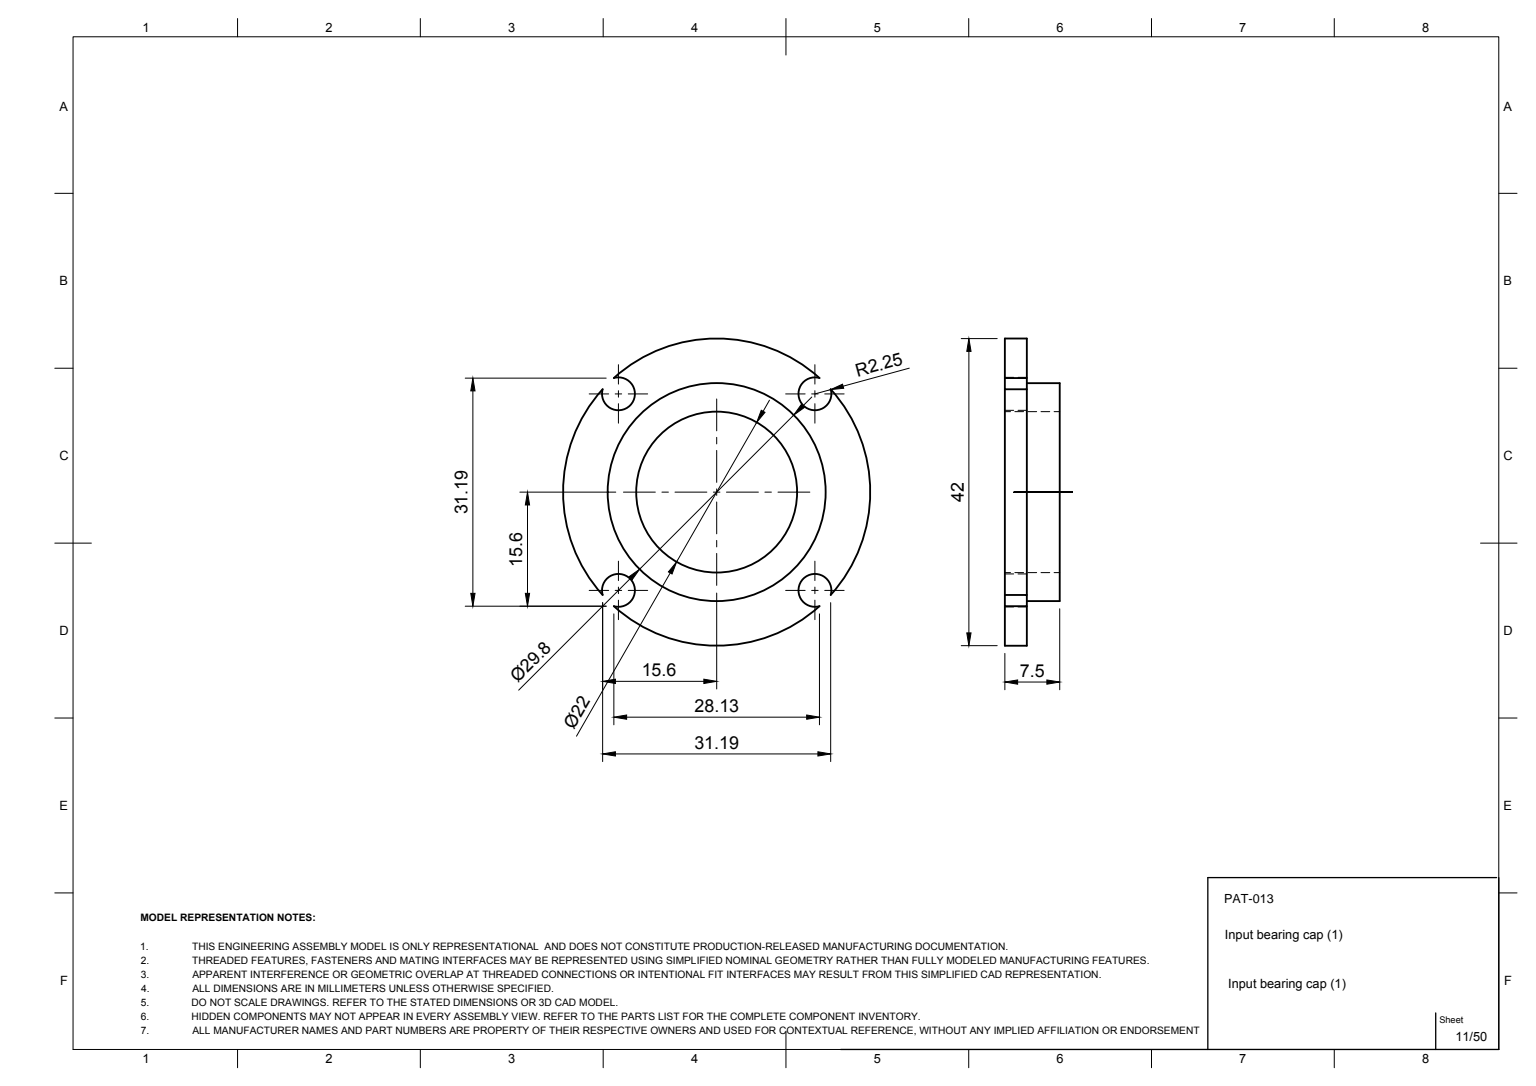
ISO-10303-21;
HEADER;
/* Generated by software containing ST-Developer
 * from STEP Tools, Inc. (www.steptools.com) 
 */

FILE_DESCRIPTION(
/* description */ ('Belt-driven linear axis on 2020 extrusion'),
/* implementation_level */ '2;1');

FILE_NAME(
/* name */ 'Input bearing cap (1).step',
/* time_stamp */ '2026-10-28T03:26:09-07:00',
/* author */ (''),
/* organization */ (''),
/* preprocessor_version */ 'ST-DEVELOPER v20.2',
/* originating_system */ 'Autodesk Translation Framework v15.17.0.0',
/* authorisation */ '');

FILE_SCHEMA (('AUTOMOTIVE_DESIGN { 1 0 10303 214 3 1 1 }'));
ENDSEC;

DATA;
#10=MECHANICAL_DESIGN_GEOMETRIC_PRESENTATION_REPRESENTATION('',(#618),#20096);
#524=SHAPE_REPRESENTATION_RELATIONSHIP('SRR','None',#20320,#570);
#570=ADVANCED_BREP_SHAPE_REPRESENTATION('',(#674),#20051);
#618=STYLED_ITEM('',(#20650),#674);
#674=MANIFOLD_SOLID_BREP('Body1',#10931);
#765=FACE_BOUND('',#2026,.T.);
#766=FACE_BOUND('',#2033,.T.);
#767=FACE_BOUND('',#2036,.T.);
#950=PLANE('',#11695);
#951=PLANE('',#11711);
#952=PLANE('',#11715);
#1352=FACE_OUTER_BOUND('',#2021,.T.);
#1353=FACE_OUTER_BOUND('',#2022,.T.);
#1354=FACE_OUTER_BOUND('',#2023,.T.);
#1355=FACE_OUTER_BOUND('',#2024,.T.);
#1356=FACE_OUTER_BOUND('',#2025,.T.);
#1357=FACE_OUTER_BOUND('',#2027,.T.);
#1358=FACE_OUTER_BOUND('',#2028,.T.);
#1359=FACE_OUTER_BOUND('',#2029,.T.);
#1360=FACE_OUTER_BOUND('',#2030,.T.);
#1361=FACE_OUTER_BOUND('',#2031,.T.);
#1362=FACE_OUTER_BOUND('',#2032,.T.);
#1363=FACE_OUTER_BOUND('',#2034,.T.);
#1364=FACE_OUTER_BOUND('',#2035,.T.);
#2021=EDGE_LOOP('',(#7667,#7668,#7669,#7670));
#2022=EDGE_LOOP('',(#7671,#7672,#7673,#7674));
#2023=EDGE_LOOP('',(#7675,#7676,#7677,#7678));
#2024=EDGE_LOOP('',(#7679,#7680,#7681,#7682));
#2025=EDGE_LOOP('',(#7683,#7684,#7685,#7686,#7687,#7688,#7689,#7690));
#2026=EDGE_LOOP('',(#7691));
#2027=EDGE_LOOP('',(#7692,#7693,#7694,#7695));
#2028=EDGE_LOOP('',(#7696,#7697,#7698,#7699));
#2029=EDGE_LOOP('',(#7700,#7701,#7702,#7703));
#2030=EDGE_LOOP('',(#7704,#7705,#7706,#7707));
#2031=EDGE_LOOP('',(#7708,#7709,#7710,#7711));
#2032=EDGE_LOOP('',(#7712));
#2033=EDGE_LOOP('',(#7713));
#2034=EDGE_LOOP('',(#7714,#7715,#7716,#7717));
#2035=EDGE_LOOP('',(#7718,#7719,#7720,#7721,#7722,#7723,#7724,#7725));
#2036=EDGE_LOOP('',(#7726));
#2790=LINE('',#16691,#3647);
#2791=LINE('',#16695,#3648);
#2792=LINE('',#16700,#3649);
#2793=LINE('',#16704,#3650);
#2794=LINE('',#16709,#3651);
#2795=LINE('',#16713,#3652);
#2796=LINE('',#16718,#3653);
#2797=LINE('',#16722,#3654);
#2798=LINE('',#16741,#3655);
#2799=LINE('',#16749,#3656);
#3647=VECTOR('',#13298,1.);
#3648=VECTOR('',#13301,1.);
#3649=VECTOR('',#13306,1.);
#3650=VECTOR('',#13309,1.);
#3651=VECTOR('',#13314,1.);
#3652=VECTOR('',#13317,1.);
#3653=VECTOR('',#13322,1.);
#3654=VECTOR('',#13325,1.);
#3655=VECTOR('',#13358,1.49);
#3656=VECTOR('',#13369,1.1);
#4461=CIRCLE('',#11684,0.225);
#4462=CIRCLE('',#11685,0.225);
#4463=CIRCLE('',#11687,0.225);
#4464=CIRCLE('',#11688,0.225);
#4465=CIRCLE('',#11690,0.225);
#4466=CIRCLE('',#11691,0.225);
#4467=CIRCLE('',#11693,0.225);
#4468=CIRCLE('',#11694,0.225);
#4469=CIRCLE('',#11696,2.1);
#4470=CIRCLE('',#11697,2.1);
#4471=CIRCLE('',#11698,2.1);
#4472=CIRCLE('',#11699,2.1);
#4473=CIRCLE('',#11700,1.49);
#4474=CIRCLE('',#11702,2.1);
#4475=CIRCLE('',#11704,2.1);
#4476=CIRCLE('',#11706,2.1);
#4477=CIRCLE('',#11708,2.1);
#4478=CIRCLE('',#11710,1.49);
#4479=CIRCLE('',#11712,1.1);
#4480=CIRCLE('',#11714,1.1);
#5030=VERTEX_POINT('',#16689);
#5031=VERTEX_POINT('',#16690);
#5032=VERTEX_POINT('',#16692);
#5033=VERTEX_POINT('',#16694);
#5034=VERTEX_POINT('',#16698);
#5035=VERTEX_POINT('',#16699);
#5036=VERTEX_POINT('',#16701);
#5037=VERTEX_POINT('',#16703);
#5038=VERTEX_POINT('',#16707);
#5039=VERTEX_POINT('',#16708);
#5040=VERTEX_POINT('',#16710);
#5041=VERTEX_POINT('',#16712);
#5042=VERTEX_POINT('',#16716);
#5043=VERTEX_POINT('',#16717);
#5044=VERTEX_POINT('',#16719);
#5045=VERTEX_POINT('',#16721);
#5046=VERTEX_POINT('',#16729);
#5047=VERTEX_POINT('',#16740);
#5048=VERTEX_POINT('',#16744);
#5049=VERTEX_POINT('',#16747);
#6048=EDGE_CURVE('',#5030,#5031,#2790,.T.);
#6049=EDGE_CURVE('',#5032,#5030,#4461,.T.);
#6050=EDGE_CURVE('',#5033,#5032,#2791,.T.);
#6051=EDGE_CURVE('',#5031,#5033,#4462,.T.);
#6052=EDGE_CURVE('',#5034,#5035,#2792,.T.);
#6053=EDGE_CURVE('',#5036,#5034,#4463,.T.);
#6054=EDGE_CURVE('',#5037,#5036,#2793,.T.);
#6055=EDGE_CURVE('',#5035,#5037,#4464,.T.);
#6056=EDGE_CURVE('',#5038,#5039,#2794,.T.);
#6057=EDGE_CURVE('',#5040,#5038,#4465,.T.);
#6058=EDGE_CURVE('',#5041,#5040,#2795,.T.);
#6059=EDGE_CURVE('',#5039,#5041,#4466,.T.);
#6060=EDGE_CURVE('',#5042,#5043,#2796,.T.);
#6061=EDGE_CURVE('',#5044,#5042,#4467,.T.);
#6062=EDGE_CURVE('',#5045,#5044,#2797,.T.);
#6063=EDGE_CURVE('',#5043,#5045,#4468,.T.);
#6064=EDGE_CURVE('',#5044,#5030,#4469,.T.);
#6065=EDGE_CURVE('',#5040,#5042,#4470,.T.);
#6066=EDGE_CURVE('',#5036,#5038,#4471,.T.);
#6067=EDGE_CURVE('',#5032,#5034,#4472,.T.);
#6068=EDGE_CURVE('',#5046,#5046,#4473,.T.);
#6069=EDGE_CURVE('',#5041,#5043,#4474,.T.);
#6070=EDGE_CURVE('',#5037,#5039,#4475,.T.);
#6071=EDGE_CURVE('',#5045,#5031,#4476,.T.);
#6072=EDGE_CURVE('',#5033,#5035,#4477,.T.);
#6073=EDGE_CURVE('',#5046,#5047,#2798,.T.);
#6074=EDGE_CURVE('',#5047,#5047,#4478,.T.);
#6075=EDGE_CURVE('',#5048,#5048,#4479,.T.);
#6076=EDGE_CURVE('',#5049,#5049,#4480,.T.);
#6077=EDGE_CURVE('',#5049,#5048,#2799,.T.);
#7667=ORIENTED_EDGE('',*,*,#6048,.F.);
#7668=ORIENTED_EDGE('',*,*,#6049,.F.);
#7669=ORIENTED_EDGE('',*,*,#6050,.F.);
#7670=ORIENTED_EDGE('',*,*,#6051,.F.);
#7671=ORIENTED_EDGE('',*,*,#6052,.F.);
#7672=ORIENTED_EDGE('',*,*,#6053,.F.);
#7673=ORIENTED_EDGE('',*,*,#6054,.F.);
#7674=ORIENTED_EDGE('',*,*,#6055,.F.);
#7675=ORIENTED_EDGE('',*,*,#6056,.F.);
#7676=ORIENTED_EDGE('',*,*,#6057,.F.);
#7677=ORIENTED_EDGE('',*,*,#6058,.F.);
#7678=ORIENTED_EDGE('',*,*,#6059,.F.);
#7679=ORIENTED_EDGE('',*,*,#6060,.F.);
#7680=ORIENTED_EDGE('',*,*,#6061,.F.);
#7681=ORIENTED_EDGE('',*,*,#6062,.F.);
#7682=ORIENTED_EDGE('',*,*,#6063,.F.);
#7683=ORIENTED_EDGE('',*,*,#6049,.T.);
#7684=ORIENTED_EDGE('',*,*,#6064,.F.);
#7685=ORIENTED_EDGE('',*,*,#6061,.T.);
#7686=ORIENTED_EDGE('',*,*,#6065,.F.);
#7687=ORIENTED_EDGE('',*,*,#6057,.T.);
#7688=ORIENTED_EDGE('',*,*,#6066,.F.);
#7689=ORIENTED_EDGE('',*,*,#6053,.T.);
#7690=ORIENTED_EDGE('',*,*,#6067,.F.);
#7691=ORIENTED_EDGE('',*,*,#6068,.T.);
#7692=ORIENTED_EDGE('',*,*,#6058,.T.);
#7693=ORIENTED_EDGE('',*,*,#6065,.T.);
#7694=ORIENTED_EDGE('',*,*,#6060,.T.);
#7695=ORIENTED_EDGE('',*,*,#6069,.F.);
#7696=ORIENTED_EDGE('',*,*,#6054,.T.);
#7697=ORIENTED_EDGE('',*,*,#6066,.T.);
#7698=ORIENTED_EDGE('',*,*,#6056,.T.);
#7699=ORIENTED_EDGE('',*,*,#6070,.F.);
#7700=ORIENTED_EDGE('',*,*,#6048,.T.);
#7701=ORIENTED_EDGE('',*,*,#6071,.F.);
#7702=ORIENTED_EDGE('',*,*,#6062,.T.);
#7703=ORIENTED_EDGE('',*,*,#6064,.T.);
#7704=ORIENTED_EDGE('',*,*,#6050,.T.);
#7705=ORIENTED_EDGE('',*,*,#6067,.T.);
#7706=ORIENTED_EDGE('',*,*,#6052,.T.);
#7707=ORIENTED_EDGE('',*,*,#6072,.F.);
#7708=ORIENTED_EDGE('',*,*,#6068,.F.);
#7709=ORIENTED_EDGE('',*,*,#6073,.T.);
#7710=ORIENTED_EDGE('',*,*,#6074,.T.);
#7711=ORIENTED_EDGE('',*,*,#6073,.F.);
#7712=ORIENTED_EDGE('',*,*,#6074,.F.);
#7713=ORIENTED_EDGE('',*,*,#6075,.F.);
#7714=ORIENTED_EDGE('',*,*,#6076,.F.);
#7715=ORIENTED_EDGE('',*,*,#6077,.T.);
#7716=ORIENTED_EDGE('',*,*,#6075,.T.);
#7717=ORIENTED_EDGE('',*,*,#6077,.F.);
#7718=ORIENTED_EDGE('',*,*,#6051,.T.);
#7719=ORIENTED_EDGE('',*,*,#6072,.T.);
#7720=ORIENTED_EDGE('',*,*,#6055,.T.);
#7721=ORIENTED_EDGE('',*,*,#6070,.T.);
#7722=ORIENTED_EDGE('',*,*,#6059,.T.);
#7723=ORIENTED_EDGE('',*,*,#6069,.T.);
#7724=ORIENTED_EDGE('',*,*,#6063,.T.);
#7725=ORIENTED_EDGE('',*,*,#6071,.T.);
#7726=ORIENTED_EDGE('',*,*,#6076,.T.);
#10118=CYLINDRICAL_SURFACE('',#11683,0.225);
#10119=CYLINDRICAL_SURFACE('',#11686,0.225);
#10120=CYLINDRICAL_SURFACE('',#11689,0.225);
#10121=CYLINDRICAL_SURFACE('',#11692,0.225);
#10122=CYLINDRICAL_SURFACE('',#11701,2.1);
#10123=CYLINDRICAL_SURFACE('',#11703,2.1);
#10124=CYLINDRICAL_SURFACE('',#11705,2.1);
#10125=CYLINDRICAL_SURFACE('',#11707,2.1);
#10126=CYLINDRICAL_SURFACE('',#11709,1.49);
#10127=CYLINDRICAL_SURFACE('',#11713,1.1);
#10403=ADVANCED_FACE('',(#1352),#10118,.F.);
#10404=ADVANCED_FACE('',(#1353),#10119,.F.);
#10405=ADVANCED_FACE('',(#1354),#10120,.F.);
#10406=ADVANCED_FACE('',(#1355),#10121,.F.);
#10407=ADVANCED_FACE('',(#1356,#765),#950,.F.);
#10408=ADVANCED_FACE('',(#1357),#10122,.T.);
#10409=ADVANCED_FACE('',(#1358),#10123,.T.);
#10410=ADVANCED_FACE('',(#1359),#10124,.T.);
#10411=ADVANCED_FACE('',(#1360),#10125,.T.);
#10412=ADVANCED_FACE('',(#1361),#10126,.T.);
#10413=ADVANCED_FACE('',(#1362,#766),#951,.F.);
#10414=ADVANCED_FACE('',(#1363),#10127,.F.);
#10415=ADVANCED_FACE('',(#1364,#767),#952,.T.);
#10931=CLOSED_SHELL('',(#10403,#10404,#10405,#10406,#10407,#10408,#10409,
#10410,#10411,#10412,#10413,#10414,#10415));
#11682=AXIS2_PLACEMENT_3D('',#16687,#13294,#13295);
#11683=AXIS2_PLACEMENT_3D('',#16688,#13296,#13297);
#11684=AXIS2_PLACEMENT_3D('',#16693,#13299,#13300);
#11685=AXIS2_PLACEMENT_3D('',#16696,#13302,#13303);
#11686=AXIS2_PLACEMENT_3D('',#16697,#13304,#13305);
#11687=AXIS2_PLACEMENT_3D('',#16702,#13307,#13308);
#11688=AXIS2_PLACEMENT_3D('',#16705,#13310,#13311);
#11689=AXIS2_PLACEMENT_3D('',#16706,#13312,#13313);
#11690=AXIS2_PLACEMENT_3D('',#16711,#13315,#13316);
#11691=AXIS2_PLACEMENT_3D('',#16714,#13318,#13319);
#11692=AXIS2_PLACEMENT_3D('',#16715,#13320,#13321);
#11693=AXIS2_PLACEMENT_3D('',#16720,#13323,#13324);
#11694=AXIS2_PLACEMENT_3D('',#16723,#13326,#13327);
#11695=AXIS2_PLACEMENT_3D('',#16724,#13328,#13329);
#11696=AXIS2_PLACEMENT_3D('',#16725,#13330,#13331);
#11697=AXIS2_PLACEMENT_3D('',#16726,#13332,#13333);
#11698=AXIS2_PLACEMENT_3D('',#16727,#13334,#13335);
#11699=AXIS2_PLACEMENT_3D('',#16728,#13336,#13337);
#11700=AXIS2_PLACEMENT_3D('',#16730,#13338,#13339);
#11701=AXIS2_PLACEMENT_3D('',#16731,#13340,#13341);
#11702=AXIS2_PLACEMENT_3D('',#16732,#13342,#13343);
#11703=AXIS2_PLACEMENT_3D('',#16733,#13344,#13345);
#11704=AXIS2_PLACEMENT_3D('',#16734,#13346,#13347);
#11705=AXIS2_PLACEMENT_3D('',#16735,#13348,#13349);
#11706=AXIS2_PLACEMENT_3D('',#16736,#13350,#13351);
#11707=AXIS2_PLACEMENT_3D('',#16737,#13352,#13353);
#11708=AXIS2_PLACEMENT_3D('',#16738,#13354,#13355);
#11709=AXIS2_PLACEMENT_3D('',#16739,#13356,#13357);
#11710=AXIS2_PLACEMENT_3D('',#16742,#13359,#13360);
#11711=AXIS2_PLACEMENT_3D('',#16743,#13361,#13362);
#11712=AXIS2_PLACEMENT_3D('',#16745,#13363,#13364);
#11713=AXIS2_PLACEMENT_3D('',#16746,#13365,#13366);
#11714=AXIS2_PLACEMENT_3D('',#16748,#13367,#13368);
#11715=AXIS2_PLACEMENT_3D('',#16750,#13370,#13371);
#13294=DIRECTION('axis',(0.,0.,1.));
#13295=DIRECTION('refdir',(1.,0.,0.));
#13296=DIRECTION('center_axis',(0.,1.,0.));
#13297=DIRECTION('ref_axis',(0.707106781186546,0.,0.707106781186549));
#13298=DIRECTION('',(0.,1.,0.));
#13299=DIRECTION('center_axis',(0.,1.,0.));
#13300=DIRECTION('ref_axis',(1.,0.,0.));
#13301=DIRECTION('',(0.,-1.,0.));
#13302=DIRECTION('center_axis',(0.,-1.,0.));
#13303=DIRECTION('ref_axis',(1.,0.,0.));
#13304=DIRECTION('center_axis',(0.,1.,0.));
#13305=DIRECTION('ref_axis',(0.707106781186547,0.,-0.707106781186548));
#13306=DIRECTION('',(0.,1.,0.));
#13307=DIRECTION('center_axis',(0.,1.,0.));
#13308=DIRECTION('ref_axis',(1.,0.,0.));
#13309=DIRECTION('',(0.,-1.,0.));
#13310=DIRECTION('center_axis',(0.,-1.,0.));
#13311=DIRECTION('ref_axis',(1.,0.,0.));
#13312=DIRECTION('center_axis',(0.,1.,0.));
#13313=DIRECTION('ref_axis',(-0.707106781186552,0.,-0.707106781186543));
#13314=DIRECTION('',(0.,1.,0.));
#13315=DIRECTION('center_axis',(0.,1.,0.));
#13316=DIRECTION('ref_axis',(1.,0.,0.));
#13317=DIRECTION('',(0.,-1.,0.));
#13318=DIRECTION('center_axis',(0.,-1.,0.));
#13319=DIRECTION('ref_axis',(1.,0.,0.));
#13320=DIRECTION('center_axis',(0.,1.,0.));
#13321=DIRECTION('ref_axis',(-0.707106781186546,0.,0.707106781186549));
#13322=DIRECTION('',(0.,1.,0.));
#13323=DIRECTION('center_axis',(0.,1.,0.));
#13324=DIRECTION('ref_axis',(1.,0.,0.));
#13325=DIRECTION('',(0.,-1.,0.));
#13326=DIRECTION('center_axis',(0.,-1.,0.));
#13327=DIRECTION('ref_axis',(1.,0.,0.));
#13328=DIRECTION('center_axis',(0.,1.,0.));
#13329=DIRECTION('ref_axis',(1.,0.,0.));
#13330=DIRECTION('center_axis',(0.,1.,0.));
#13331=DIRECTION('ref_axis',(1.,0.,0.));
#13332=DIRECTION('center_axis',(0.,1.,0.));
#13333=DIRECTION('ref_axis',(1.,0.,0.));
#13334=DIRECTION('center_axis',(0.,1.,0.));
#13335=DIRECTION('ref_axis',(1.,0.,0.));
#13336=DIRECTION('center_axis',(0.,1.,0.));
#13337=DIRECTION('ref_axis',(1.,0.,0.));
#13338=DIRECTION('center_axis',(0.,1.,0.));
#13339=DIRECTION('ref_axis',(1.,0.,0.));
#13340=DIRECTION('center_axis',(0.,1.,0.));
#13341=DIRECTION('ref_axis',(1.,0.,0.));
#13342=DIRECTION('center_axis',(0.,1.,0.));
#13343=DIRECTION('ref_axis',(1.,0.,0.));
#13344=DIRECTION('center_axis',(0.,1.,0.));
#13345=DIRECTION('ref_axis',(1.,0.,0.));
#13346=DIRECTION('center_axis',(0.,1.,0.));
#13347=DIRECTION('ref_axis',(1.,0.,0.));
#13348=DIRECTION('center_axis',(0.,1.,0.));
#13349=DIRECTION('ref_axis',(1.,0.,0.));
#13350=DIRECTION('center_axis',(0.,1.,0.));
#13351=DIRECTION('ref_axis',(1.,0.,0.));
#13352=DIRECTION('center_axis',(0.,1.,0.));
#13353=DIRECTION('ref_axis',(-1.,0.,-1.22464679914735E-16));
#13354=DIRECTION('center_axis',(0.,1.,0.));
#13355=DIRECTION('ref_axis',(1.,0.,0.));
#13356=DIRECTION('center_axis',(0.,1.,0.));
#13357=DIRECTION('ref_axis',(1.,0.,0.));
#13358=DIRECTION('',(0.,-1.,0.));
#13359=DIRECTION('center_axis',(0.,1.,0.));
#13360=DIRECTION('ref_axis',(1.,0.,0.));
#13361=DIRECTION('center_axis',(0.,1.,0.));
#13362=DIRECTION('ref_axis',(1.,0.,0.));
#13363=DIRECTION('center_axis',(0.,-1.,0.));
#13364=DIRECTION('ref_axis',(1.,0.,0.));
#13365=DIRECTION('center_axis',(0.,1.,0.));
#13366=DIRECTION('ref_axis',(1.,0.,0.));
#13367=DIRECTION('center_axis',(0.,-1.,0.));
#13368=DIRECTION('ref_axis',(1.,0.,0.));
#13369=DIRECTION('',(0.,-1.,0.));
#13370=DIRECTION('center_axis',(0.,1.,0.));
#13371=DIRECTION('ref_axis',(1.,0.,0.));
#16687=CARTESIAN_POINT('',(0.,0.,0.));
#16688=CARTESIAN_POINT('Origin',(-1.34350288425444,1.7,5.65649711574556));
#16689=CARTESIAN_POINT('',(-1.40634555589641,1.8,5.4404512904656));
#16690=CARTESIAN_POINT('',(-1.40634555589641,2.1,5.4404512904656));
#16691=CARTESIAN_POINT('',(-1.40634555589641,1.7,5.4404512904656));
#16692=CARTESIAN_POINT('',(-1.5595487095344,1.8,5.59365444410359));
#16693=CARTESIAN_POINT('Origin',(-1.34350288425444,1.8,5.65649711574556));
#16694=CARTESIAN_POINT('',(-1.5595487095344,2.1,5.59365444410359));
#16695=CARTESIAN_POINT('',(-1.5595487095344,1.7,5.59365444410359));
#16696=CARTESIAN_POINT('Origin',(-1.34350288425444,2.1,5.65649711574556));
#16697=CARTESIAN_POINT('Origin',(-1.34350288425444,1.7,8.34350288425444));
#16698=CARTESIAN_POINT('',(-1.5595487095344,1.8,8.40634555589641));
#16699=CARTESIAN_POINT('',(-1.5595487095344,2.1,8.40634555589641));
#16700=CARTESIAN_POINT('',(-1.5595487095344,1.7,8.40634555589641));
#16701=CARTESIAN_POINT('',(-1.40634555589641,1.8,8.5595487095344));
#16702=CARTESIAN_POINT('Origin',(-1.34350288425444,1.8,8.34350288425444));
#16703=CARTESIAN_POINT('',(-1.40634555589641,2.1,8.5595487095344));
#16704=CARTESIAN_POINT('',(-1.40634555589641,1.7,8.5595487095344));
#16705=CARTESIAN_POINT('Origin',(-1.34350288425444,2.1,8.34350288425444));
#16706=CARTESIAN_POINT('Origin',(1.34350288425444,1.7,8.34350288425444));
#16707=CARTESIAN_POINT('',(1.40634555589641,1.8,8.5595487095344));
#16708=CARTESIAN_POINT('',(1.40634555589641,2.1,8.5595487095344));
#16709=CARTESIAN_POINT('',(1.40634555589641,1.7,8.5595487095344));
#16710=CARTESIAN_POINT('',(1.5595487095344,1.8,8.40634555589641));
#16711=CARTESIAN_POINT('Origin',(1.34350288425444,1.8,8.34350288425444));
#16712=CARTESIAN_POINT('',(1.5595487095344,2.1,8.40634555589641));
#16713=CARTESIAN_POINT('',(1.5595487095344,1.7,8.40634555589641));
#16714=CARTESIAN_POINT('Origin',(1.34350288425444,2.1,8.34350288425444));
#16715=CARTESIAN_POINT('Origin',(1.34350288425444,1.7,5.65649711574556));
#16716=CARTESIAN_POINT('',(1.5595487095344,1.8,5.59365444410359));
#16717=CARTESIAN_POINT('',(1.5595487095344,2.1,5.59365444410359));
#16718=CARTESIAN_POINT('',(1.5595487095344,1.7,5.59365444410359));
#16719=CARTESIAN_POINT('',(1.40634555589641,1.8,5.4404512904656));
#16720=CARTESIAN_POINT('Origin',(1.34350288425444,1.8,5.65649711574556));
#16721=CARTESIAN_POINT('',(1.40634555589641,2.1,5.4404512904656));
#16722=CARTESIAN_POINT('',(1.40634555589641,1.7,5.4404512904656));
#16723=CARTESIAN_POINT('Origin',(1.34350288425444,2.1,5.65649711574556));
#16724=CARTESIAN_POINT('Origin',(0.,1.8,7.));
#16725=CARTESIAN_POINT('Origin',(0.,1.8,7.));
#16726=CARTESIAN_POINT('Origin',(0.,1.8,7.));
#16727=CARTESIAN_POINT('Origin',(0.,1.8,7.));
#16728=CARTESIAN_POINT('Origin',(0.,1.8,7.));
#16729=CARTESIAN_POINT('',(-1.49,1.8,7.));
#16730=CARTESIAN_POINT('Origin',(0.,1.8,7.));
#16731=CARTESIAN_POINT('Origin',(0.,1.8,7.));
#16732=CARTESIAN_POINT('Origin',(0.,2.1,7.));
#16733=CARTESIAN_POINT('Origin',(0.,1.8,7.));
#16734=CARTESIAN_POINT('Origin',(0.,2.1,7.));
#16735=CARTESIAN_POINT('Origin',(0.,1.8,7.));
#16736=CARTESIAN_POINT('Origin',(0.,2.1,7.));
#16737=CARTESIAN_POINT('Origin',(0.,1.8,7.));
#16738=CARTESIAN_POINT('Origin',(0.,2.1,7.));
#16739=CARTESIAN_POINT('Origin',(0.,1.35,7.));
#16740=CARTESIAN_POINT('',(-1.49,1.35,7.));
#16741=CARTESIAN_POINT('',(-1.49,1.35,7.));
#16742=CARTESIAN_POINT('Origin',(0.,1.35,7.));
#16743=CARTESIAN_POINT('Origin',(0.,1.35,7.));
#16744=CARTESIAN_POINT('',(-1.1,1.35,7.));
#16745=CARTESIAN_POINT('Origin',(0.,1.35,7.));
#16746=CARTESIAN_POINT('Origin',(0.,1.8,7.));
#16747=CARTESIAN_POINT('',(-1.1,2.1,7.));
#16748=CARTESIAN_POINT('Origin',(0.,2.1,7.));
#16749=CARTESIAN_POINT('',(-1.1,1.8,7.));
#16750=CARTESIAN_POINT('Origin',(0.,2.1,7.));
#19997=UNCERTAINTY_MEASURE_WITH_UNIT(LENGTH_MEASURE(0.001),#20097,
'DISTANCE_ACCURACY_VALUE',
'Maximum model space distance between geometric entities at asserted c
onnectivities');
#20042=UNCERTAINTY_MEASURE_WITH_UNIT(LENGTH_MEASURE(0.001),#20097,
'DISTANCE_ACCURACY_VALUE',
'Maximum model space distance between geometric entities at asserted c
onnectivities');
#20051=(
GEOMETRIC_REPRESENTATION_CONTEXT(3)
GLOBAL_UNCERTAINTY_ASSIGNED_CONTEXT((#19997))
GLOBAL_UNIT_ASSIGNED_CONTEXT((#20097,#20099,#20100))
REPRESENTATION_CONTEXT('','3D')
);
#20096=(
GEOMETRIC_REPRESENTATION_CONTEXT(3)
GLOBAL_UNCERTAINTY_ASSIGNED_CONTEXT((#20042))
GLOBAL_UNIT_ASSIGNED_CONTEXT((#20097,#20099,#20100))
REPRESENTATION_CONTEXT('','3D')
);
#20097=(
LENGTH_UNIT()
NAMED_UNIT(*)
SI_UNIT(.CENTI.,.METRE.)
);
#20099=(
NAMED_UNIT(*)
PLANE_ANGLE_UNIT()
SI_UNIT($,.RADIAN.)
);
#20100=(
NAMED_UNIT(*)
SI_UNIT($,.STERADIAN.)
SOLID_ANGLE_UNIT()
);
#20109=SHAPE_DEFINITION_REPRESENTATION(#20162,#20320);
#20162=PRODUCT_DEFINITION_SHAPE('',$,#20374);
#20320=SHAPE_REPRESENTATION('',(#11682),#20051);
#20365=PRODUCT_DEFINITION_CONTEXT('part definition',#20526,'design');
#20374=PRODUCT_DEFINITION('Input bearing cap (1)','Input bearing cap (1)',
#20427,#20365);
#20427=PRODUCT_DEFINITION_FORMATION('',$,#20536);
#20526=APPLICATION_CONTEXT(
'Core Data for Automotive Mechanical Design Process');
#20527=PRODUCT_CONTEXT('part definition',#20526,'mechanical');
#20536=PRODUCT('Input bearing cap (1)','Input bearing cap (1)',
'Input bearing cap (1)',(#20527));
#20644=COLOUR_RGB('Grey',0.48,0.52,0.57);
#20645=FILL_AREA_STYLE_COLOUR('',#20644);
#20646=FILL_AREA_STYLE('',(#20645));
#20647=SURFACE_STYLE_FILL_AREA(#20646);
#20648=SURFACE_SIDE_STYLE('',(#20647));
#20649=SURFACE_STYLE_USAGE(.BOTH.,#20648);
#20650=PRESENTATION_STYLE_ASSIGNMENT((#20649));
ENDSEC;
END-ISO-10303-21;
